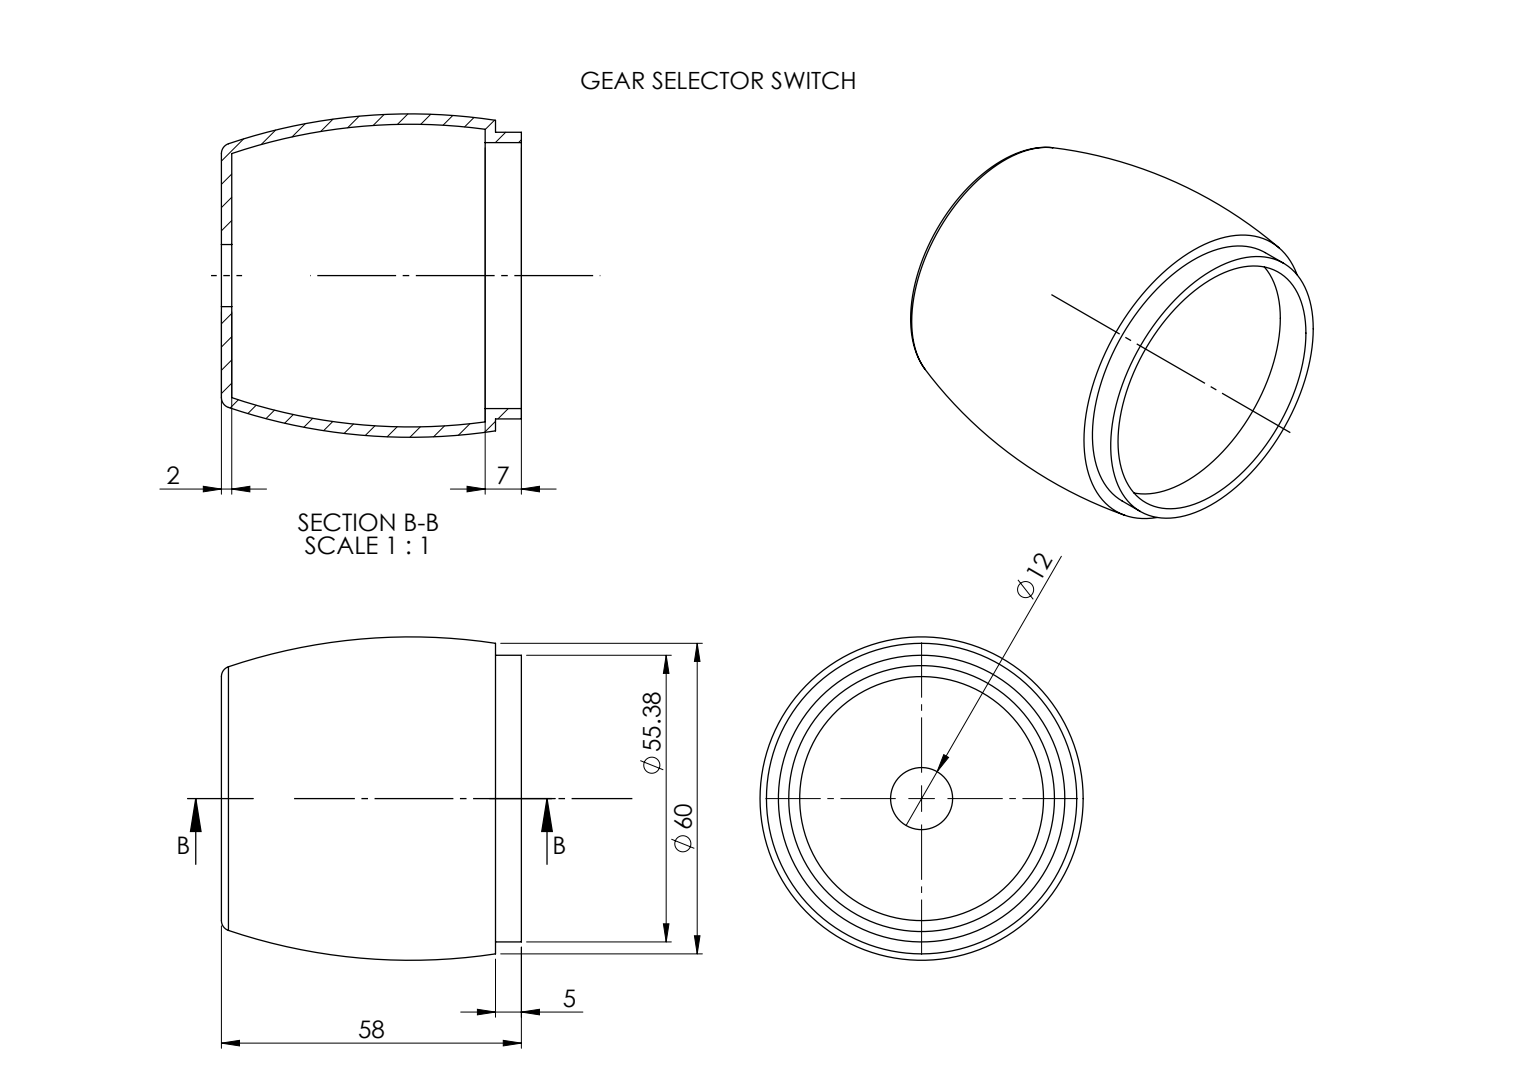
ISO-10303-21;
HEADER;
FILE_DESCRIPTION (('STEP AP214'),
    '1' );
FILE_NAME ('gear selector switch.step',
    '2026-10-05T20:22:16',
    ( '' ),
    ( '' ),
    'SwSTEP 2.0',
    'SolidWorks 2026',
    '' );
FILE_SCHEMA (( 'AUTOMOTIVE_DESIGN' ));
ENDSEC;

DATA;
#4=DIRECTION ( 'NONE',  ( 0.000000000000000000, 0.000000000000000000, -1.000000000000000000 ) ) ;
#45=ORIENTED_EDGE ( 'NONE', *, *, #7953, .F. ) ;
#49=PRODUCT_DEFINITION ( 'UNKNOWN', '', #15196, #232 ) ;
#123=PLANE ( 'NONE',  #15795 ) ;
#134=VERTEX_POINT ( 'NONE', #6129 ) ;
#138=ADVANCED_FACE ( 'NONE', ( #7376, #14017 ), #15677, .T. ) ;
#146=EDGE_CURVE ( 'NONE', #17383, #9593, #6108, .T. ) ;
#205=LINE ( 'NONE', #13586, #10347 ) ;
#217=SHAPE_DEFINITION_REPRESENTATION ( #9683, #10772 ) ;
#232=PRODUCT_DEFINITION_CONTEXT ( 'detailed design', #10711, 'design' ) ;
#249=FILL_AREA_STYLE_COLOUR ( '', #15123 ) ;
#272=CIRCLE ( 'NONE', #13562, 28.26633746182136164 ) ;
#285=DIRECTION ( 'NONE',  ( 0.000000000000000000, 0.000000000000000000, -1.000000000000000000 ) ) ;
#287=CIRCLE ( 'NONE', #5084, 23.57392898041429774 ) ;
#308=PLANE ( 'NONE',  #8782 ) ;
#348=CARTESIAN_POINT ( 'NONE',  ( -116.4755503550297107, 171.6227766016838245, 0.000000000000000000 ) ) ;
#409=AXIS2_PLACEMENT_3D ( 'NONE', #3562, #17022, #2059 ) ;
#411=ORIENTED_EDGE ( 'NONE', *, *, #16163, .T. ) ;
#425=ADVANCED_FACE ( 'NONE', ( #5501 ), #4977, .T. ) ;
#430=MECHANICAL_DESIGN_GEOMETRIC_PRESENTATION_REPRESENTATION('',(#7494),#12593);
#459=CARTESIAN_POINT ( 'NONE',  ( -95.00000000000000000, 171.6227766016838245, 0.000000000000000000 ) ) ;
#475=AXIS2_PLACEMENT_3D ( 'NONE', #11596, #1866, #6196 ) ;
#499=EDGE_CURVE ( 'NONE', #9593, #12318, #8101, .T. ) ;
#514=CYLINDRICAL_SURFACE ( 'NONE', #16412, 6.000000000000005329 ) ;
#554=VERTEX_POINT ( 'NONE', #15318 ) ;
#641=CARTESIAN_POINT ( 'NONE',  ( -153.0000000000000284, 171.6227766016838245, 0.000000000000000000 ) ) ;
#646=DIRECTION ( 'NONE',  ( 0.000000000000000000, 0.000000000000000000, 1.000000000000000000 ) ) ;
#675=SHAPE_REPRESENTATION_RELATIONSHIP ( 'NONE' , 'NONE' ,  #10772, #1721 ) ;
#691=CARTESIAN_POINT ( 'NONE',  ( -103.0000000000000142, 171.6227766016838245, 0.000000000000000000 ) ) ;
#724=CARTESIAN_POINT ( 'NONE',  ( -102.0000000000000142, 201.6227766016838245, 0.000000000000000000 ) ) ;
#743=AXIS2_PLACEMENT_3D ( 'NONE', #8605, #17020, #646 ) ;
#785=AXIS2_PLACEMENT_3D ( 'NONE', #9707, #16108, #10859 ) ;
#787=VECTOR ( 'NONE', #3451, 1000.000000000000000 ) ;
#893=ADVANCED_FACE ( 'NONE', ( #4594 ), #514, .F. ) ;
#959=ORIENTED_EDGE ( 'NONE', *, *, #13344, .T. ) ;
#972=DIRECTION ( 'NONE',  ( -0.000000000000000000, 0.000000000000000000, -1.000000000000000000 ) ) ;
#985=AXIS2_PLACEMENT_3D ( 'NONE', #17428, #10947, #13359 ) ;
#996=ORIENTED_EDGE ( 'NONE', *, *, #2991, .F. ) ;
#1026=TOROIDAL_SURFACE ( 'NONE', #8943, -78.75916623668499028, 108.0000000000000142 ) ;
#1028=CIRCLE ( 'NONE', #3301, 2.000000000000001776 ) ;
#1036=VERTEX_POINT ( 'NONE', #6706 ) ;
#1137=ORIENTED_EDGE ( 'NONE', *, *, #8044, .F. ) ;
#1138=CARTESIAN_POINT ( 'NONE',  ( -103.0000000000000142, 171.6227766016838245, 0.000000000000000000 ) ) ;
#1225=FACE_OUTER_BOUND ( 'NONE', #4522, .T. ) ;
#1270=AXIS2_PLACEMENT_3D ( 'NONE', #12415, #2602, #285 ) ;
#1280=PRODUCT_CONTEXT ( 'NONE', #3711, 'mechanical' ) ;
#1401=ADVANCED_FACE ( 'NONE', ( #15134 ), #11070, .F. ) ;
#1454=EDGE_CURVE ( 'NONE', #12318, #9593, #272, .T. ) ;
#1559=LINE ( 'NONE', #6964, #4454 ) ;
#1613=FACE_OUTER_BOUND ( 'NONE', #14014, .T. ) ;
#1631=VECTOR ( 'NONE', #13356, 1000.000000000000000 ) ;
#1699=DIRECTION ( 'NONE',  ( 0.000000000000000000, 0.000000000000000000, -1.000000000000000000 ) ) ;
#1707=PLANE ( 'NONE',  #14282 ) ;
#1714=CARTESIAN_POINT ( 'NONE',  ( -151.0000000000000284, 171.6227766016838245, 0.000000000000000000 ) ) ;
#1721=ADVANCED_BREP_SHAPE_REPRESENTATION ( '', ( #11363, #3583 ), #3025 ) ;
#1767=DIRECTION ( 'NONE',  ( 0.000000000000000000, 0.000000000000000000, -1.000000000000000000 ) ) ;
#1821=ORIENTED_EDGE ( 'NONE', *, *, #14197, .T. ) ;
#1836=PRESENTATION_STYLE_ASSIGNMENT (( #11217 ) ) ;
#1866=DIRECTION ( 'NONE',  ( 1.000000000000000000, -0.000000000000000000, -0.000000000000000000 ) ) ;
#1867=ADVANCED_FACE ( 'NONE', ( #5019, #10412 ), #123, .T. ) ;
#1901=CARTESIAN_POINT ( 'NONE',  ( -103.0000000000000142, 171.6227766016838245, 25.69059892324149175 ) ) ;
#1911=ORIENTED_EDGE ( 'NONE', *, *, #8044, .T. ) ;
#1914=FILL_AREA_STYLE_COLOUR ( '', #12928 ) ;
#1994=ORIENTED_EDGE ( 'NONE', *, *, #13315, .T. ) ;
#2031=CARTESIAN_POINT ( 'NONE',  ( -95.00000000000000000, 171.6227766016838245, 27.69059892324149530 ) ) ;
#2035=ORIENTED_EDGE ( 'NONE', *, *, #16198, .F. ) ;
#2059=DIRECTION ( 'NONE',  ( 0.000000000000000000, 0.000000000000000000, 1.000000000000000000 ) ) ;
#2068=DIRECTION ( 'NONE',  ( 0.000000000000000000, 0.000000000000000000, -1.000000000000000000 ) ) ;
#2111=CIRCLE ( 'NONE', #5222, 108.0000000000000142 ) ;
#2139=DIRECTION ( 'NONE',  ( -1.000000000000000000, 0.000000000000000000, 0.000000000000000000 ) ) ;
#2177=CARTESIAN_POINT ( 'NONE',  ( -95.00000000000000000, 171.6227766016838245, -25.69059892324149175 ) ) ;
#2190=CARTESIAN_POINT ( 'NONE',  ( -103.0000000000000142, 171.6227766016838245, -25.69059892324149175 ) ) ;
#2191=AXIS2_PLACEMENT_3D ( 'NONE', #4347, #13833, #1699 ) ;
#2195=VERTEX_POINT ( 'NONE', #9129 ) ;
#2227=DIRECTION ( 'NONE',  ( 0.000000000000000000, 0.000000000000000000, 1.000000000000000000 ) ) ;
#2275=EDGE_LOOP ( 'NONE', ( #10294, #17016, #12234, #9716 ) ) ;
#2291=VERTEX_POINT ( 'NONE', #16146 ) ;
#2361=ORIENTED_EDGE ( 'NONE', *, *, #7591, .T. ) ;
#2375=TOROIDAL_SURFACE ( 'NONE', #9156, -78.75916623668499028, 110.0000000000000142 ) ;
#2446=CIRCLE ( 'NONE', #14895, 27.69059892324149530 ) ;
#2461=STYLED_ITEM ( 'NONE', ( #16877 ), #1721 ) ;
#2472=AXIS2_PLACEMENT_3D ( 'NONE', #5028, #10419, #9274 ) ;
#2501=CIRCLE ( 'NONE', #10408, 6.000000000000005329 ) ;
#2600=ORIENTED_EDGE ( 'NONE', *, *, #3605, .T. ) ;
#2602=DIRECTION ( 'NONE',  ( 1.000000000000000000, -0.000000000000000000, -0.000000000000000000 ) ) ;
#2682=DIRECTION ( 'NONE',  ( 0.000000000000000000, 0.000000000000000000, -1.000000000000000000 ) ) ;
#2721=( NAMED_UNIT ( * ) SI_UNIT ( $, .STERADIAN. ) SOLID_ANGLE_UNIT ( ) );
#2726=EDGE_CURVE ( 'NONE', #5242, #10626, #4773, .T. ) ;
#2737=DIRECTION ( 'NONE',  ( 0.000000000000000000, 0.000000000000000000, -1.000000000000000000 ) ) ;
#2763=EDGE_LOOP ( 'NONE', ( #17460, #14468, #9016, #6481 ) ) ;
#2816=AXIS2_PLACEMENT_3D ( 'NONE', #9799, #14938, #5735 ) ;
#2846=ADVANCED_FACE ( 'NONE', ( #15997 ), #8199, .T. ) ;
#2855=CYLINDRICAL_SURFACE ( 'NONE', #1270, 6.000000000000005329 ) ;
#2928=ORIENTED_EDGE ( 'NONE', *, *, #2726, .T. ) ;
#2942=ORIENTED_EDGE ( 'NONE', *, *, #16368, .F. ) ;
#2991=EDGE_CURVE ( 'NONE', #15814, #10603, #9332, .T. ) ;
#3014=DIRECTION ( 'NONE',  ( 0.000000000000000000, 0.000000000000000000, -1.000000000000000000 ) ) ;
#3021=CARTESIAN_POINT ( 'NONE',  ( -100.0000000000000000, 171.6227766016838245, 0.000000000000000000 ) ) ;
#3025=( GEOMETRIC_REPRESENTATION_CONTEXT ( 3 ) GLOBAL_UNCERTAINTY_ASSIGNED_CONTEXT ( ( #7361 ) ) GLOBAL_UNIT_ASSIGNED_CONTEXT ( ( #7140, #5383, #2721 ) ) REPRESENTATION_CONTEXT ( 'NONE', 'WORKASPACE' ) );
#3197=PRODUCT ( 'gear selector switch', 'gear selector switch', '', ( #1280 ) ) ;
#3233=CIRCLE ( 'NONE', #409, 23.57392898041431195 ) ;
#3301=AXIS2_PLACEMENT_3D ( 'NONE', #3612, #10794, #2737 ) ;
#3322=EDGE_CURVE ( 'NONE', #8608, #3610, #10467, .T. ) ;
#3356=ORIENTED_EDGE ( 'NONE', *, *, #7036, .F. ) ;
#3357=DIRECTION ( 'NONE',  ( 1.000000000000000000, -0.000000000000000000, -0.000000000000000000 ) ) ;
#3408=DIRECTION ( 'NONE',  ( 1.000000000000000000, -0.000000000000000000, -0.000000000000000000 ) ) ;
#3414=DIRECTION ( 'NONE',  ( -1.000000000000000000, 0.000000000000000000, 0.000000000000000000 ) ) ;
#3423=ADVANCED_FACE ( 'NONE', ( #5710, #10918 ), #308, .F. ) ;
#3451=DIRECTION ( 'NONE',  ( 1.000000000000000000, -0.000000000000000000, -0.000000000000000000 ) ) ;
#3522=AXIS2_PLACEMENT_3D ( 'NONE', #9734, #5760, #3014 ) ;
#3562=CARTESIAN_POINT ( 'NONE',  ( -153.0000000000000284, 171.6227766016838245, 0.000000000000000000 ) ) ;
#3583=AXIS2_PLACEMENT_3D ( 'NONE', #5482, #6893, #8222 ) ;
#3605=EDGE_CURVE ( 'NONE', #1036, #16730, #8421, .T. ) ;
#3610=VERTEX_POINT ( 'NONE', #7874 ) ;
#3612=CARTESIAN_POINT ( 'NONE',  ( -151.0000000000000284, 171.6227766016838245, 23.57392898041431195 ) ) ;
#3641=CARTESIAN_POINT ( 'NONE',  ( -100.0000000000000000, 171.6227766016838245, 30.00000000000000711 ) ) ;
#3711=APPLICATION_CONTEXT ( 'automotive_design' ) ;
#3712=DIRECTION ( 'NONE',  ( 1.000000000000000000, -0.000000000000000000, -0.000000000000000000 ) ) ;
#3756=EDGE_LOOP ( 'NONE', ( #14052, #411 ) ) ;
#3813=CARTESIAN_POINT ( 'NONE',  ( -103.0000000000000142, 171.6227766016838245, 0.000000000000000000 ) ) ;
#3889=DIRECTION ( 'NONE',  ( 1.000000000000000000, -0.000000000000000000, -0.000000000000000000 ) ) ;
#3895=AXIS2_PLACEMENT_3D ( 'NONE', #1138, #3889, #14500 ) ;
#4041=CARTESIAN_POINT ( 'NONE',  ( -116.4755503550297107, 171.6227766016838245, 78.75916623668499028 ) ) ;
#4069=ORIENTED_EDGE ( 'NONE', *, *, #5991, .T. ) ;
#4091=DIRECTION ( 'NONE',  ( 0.000000000000000000, 0.000000000000000000, -1.000000000000000000 ) ) ;
#4106=ORIENTED_EDGE ( 'NONE', *, *, #16368, .T. ) ;
#4108=DIRECTION ( 'NONE',  ( 1.000000000000000000, -0.000000000000000000, -0.000000000000000000 ) ) ;
#4111=ORIENTED_EDGE ( 'NONE', *, *, #13315, .F. ) ;
#4129=EDGE_LOOP ( 'NONE', ( #4653, #5827 ) ) ;
#4176=DIRECTION ( 'NONE',  ( 1.000000000000000000, -0.000000000000000000, -0.000000000000000000 ) ) ;
#4209=DIRECTION ( 'NONE',  ( 0.000000000000000000, 0.000000000000000000, 1.000000000000000000 ) ) ;
#4267=DIRECTION ( 'NONE',  ( 0.000000000000000000, 0.000000000000000000, -1.000000000000000000 ) ) ;
#4268=EDGE_LOOP ( 'NONE', ( #12681, #16145 ) ) ;
#4347=CARTESIAN_POINT ( 'NONE',  ( -103.0000000000000142, 171.6227766016838245, 0.000000000000000000 ) ) ;
#4354=AXIS2_PLACEMENT_3D ( 'NONE', #4478, #3408, #2068 ) ;
#4361=DIRECTION ( 'NONE',  ( 0.000000000000000000, 0.000000000000000000, -1.000000000000000000 ) ) ;
#4363=ORIENTED_EDGE ( 'NONE', *, *, #146, .F. ) ;
#4454=VECTOR ( 'NONE', #12364, 1000.000000000000000 ) ;
#4478=CARTESIAN_POINT ( 'NONE',  ( -95.00000000000000000, 171.6227766016838245, 0.000000000000000000 ) ) ;
#4522=EDGE_LOOP ( 'NONE', ( #13245, #15418, #16764, #6931 ) ) ;
#4540=DIRECTION ( 'NONE',  ( 1.000000000000000000, -0.000000000000000000, -0.000000000000000000 ) ) ;
#4541=CIRCLE ( 'NONE', #5390, 110.0000000000000142 ) ;
#4594=FACE_OUTER_BOUND ( 'NONE', #16314, .T. ) ;
#4615=DIRECTION ( 'NONE',  ( 1.000000000000000000, -0.000000000000000000, -0.000000000000000000 ) ) ;
#4653=ORIENTED_EDGE ( 'NONE', *, *, #10399, .T. ) ;
#4702=AXIS2_PLACEMENT_3D ( 'NONE', #10035, #3414, #16785 ) ;
#4739=FACE_BOUND ( 'NONE', #6262, .T. ) ;
#4768=ORIENTED_EDGE ( 'NONE', *, *, #15114, .T. ) ;
#4769=DIRECTION ( 'NONE',  ( 1.000000000000000000, -0.000000000000000000, -0.000000000000000000 ) ) ;
#4773=LINE ( 'NONE', #2190, #16125 ) ;
#4778=CIRCLE ( 'NONE', #5347, 30.00000000000000000 ) ;
#4834=ORIENTED_EDGE ( 'NONE', *, *, #10792, .F. ) ;
#4845=ADVANCED_FACE ( 'NONE', ( #5510 ), #2855, .F. ) ;
#4848=CARTESIAN_POINT ( 'NONE',  ( -116.4755503550297107, 171.6227766016838245, -78.75916623668499028 ) ) ;
#4854=DIRECTION ( 'NONE',  ( 0.000000000000000000, 0.000000000000000000, -1.000000000000000000 ) ) ;
#4914=CARTESIAN_POINT ( 'NONE',  ( -153.0000000000000284, 171.6227766016838245, 6.000000000000005329 ) ) ;
#4925=EDGE_CURVE ( 'NONE', #2195, #554, #10302, .T. ) ;
#4977=TOROIDAL_SURFACE ( 'NONE', #9498, -78.75916623668499028, 110.0000000000000142 ) ;
#4996=ADVANCED_FACE ( 'NONE', ( #11347, #7365 ), #1707, .F. ) ;
#5019=FACE_OUTER_BOUND ( 'NONE', #8020, .T. ) ;
#5028=CARTESIAN_POINT ( 'NONE',  ( -102.0000000000000142, 171.6227766016838245, 0.000000000000000000 ) ) ;
#5084=AXIS2_PLACEMENT_3D ( 'NONE', #16995, #3712, #9096 ) ;
#5121=VERTEX_POINT ( 'NONE', #3641 ) ;
#5127=DIRECTION ( 'NONE',  ( 0.000000000000000000, 0.000000000000000000, -1.000000000000000000 ) ) ;
#5146=DIRECTION ( 'NONE',  ( 1.000000000000000000, -0.000000000000000000, -0.000000000000000000 ) ) ;
#5171=EDGE_LOOP ( 'NONE', ( #6592, #2361, #16013, #15183 ) ) ;
#5222=AXIS2_PLACEMENT_3D ( 'NONE', #12160, #8164, #12417 ) ;
#5242=VERTEX_POINT ( 'NONE', #12013 ) ;
#5246=VERTEX_POINT ( 'NONE', #17147 ) ;
#5302=DIRECTION ( 'NONE',  ( 1.000000000000000000, -0.000000000000000000, -0.000000000000000000 ) ) ;
#5347=AXIS2_PLACEMENT_3D ( 'NONE', #12562, #16738, #9906 ) ;
#5383=( NAMED_UNIT ( * ) PLANE_ANGLE_UNIT ( ) SI_UNIT ( $, .RADIAN. ) );
#5390=AXIS2_PLACEMENT_3D ( 'NONE', #4848, #14229, #7578 ) ;
#5482=CARTESIAN_POINT ( 'NONE',  ( 0.000000000000000000, 0.000000000000000000, 0.000000000000000000 ) ) ;
#5501=FACE_OUTER_BOUND ( 'NONE', #5171, .T. ) ;
#5510=FACE_OUTER_BOUND ( 'NONE', #9230, .T. ) ;
#5520=DIRECTION ( 'NONE',  ( 0.000000000000000000, 0.000000000000000000, -1.000000000000000000 ) ) ;
#5560=CARTESIAN_POINT ( 'NONE',  ( -95.00000000000000000, 171.6227766016838245, 25.69059892324149175 ) ) ;
#5563=FILL_AREA_STYLE ('',( #249 ) ) ;
#5644=DIRECTION ( 'NONE',  ( 1.000000000000000000, -0.000000000000000000, -0.000000000000000000 ) ) ;
#5710=FACE_BOUND ( 'NONE', #4268, .T. ) ;
#5735=DIRECTION ( 'NONE',  ( 0.000000000000000000, 0.000000000000000000, -1.000000000000000000 ) ) ;
#5760=DIRECTION ( 'NONE',  ( 1.000000000000000000, -0.000000000000000000, -0.000000000000000000 ) ) ;
#5827=ORIENTED_EDGE ( 'NONE', *, *, #2991, .T. ) ;
#5897=ORIENTED_EDGE ( 'NONE', *, *, #14197, .F. ) ;
#5912=CARTESIAN_POINT ( 'NONE',  ( -153.0000000000000284, 171.6227766016838245, -6.000000000000005329 ) ) ;
#5968=CARTESIAN_POINT ( 'NONE',  ( -151.0000000000000284, 171.6227766016838245, -23.57392898041431195 ) ) ;
#5985=FACE_OUTER_BOUND ( 'NONE', #10484, .T. ) ;
#5991=EDGE_CURVE ( 'NONE', #17383, #134, #15147, .T. ) ;
#5994=ORIENTED_EDGE ( 'NONE', *, *, #7134, .T. ) ;
#6034=ADVANCED_FACE ( 'NONE', ( #1613 ), #1026, .F. ) ;
#6085=DIRECTION ( 'NONE',  ( 0.000000000000000000, 0.000000000000000000, -1.000000000000000000 ) ) ;
#6108=CIRCLE ( 'NONE', #743, 108.0000000000000142 ) ;
#6117=DIRECTION ( 'NONE',  ( 1.000000000000000000, 0.000000000000000000, -0.000000000000000000 ) ) ;
#6129=CARTESIAN_POINT ( 'NONE',  ( -151.0000000000000284, 171.6227766016838245, -23.57392898041429774 ) ) ;
#6153=CIRCLE ( 'NONE', #2472, 25.69059892324149175 ) ;
#6177=CARTESIAN_POINT ( 'NONE',  ( -95.00000000000000000, 171.6227766016838245, 0.000000000000000000 ) ) ;
#6196=DIRECTION ( 'NONE',  ( 0.000000000000000000, 0.000000000000000000, -1.000000000000000000 ) ) ;
#6214=ADVANCED_FACE ( 'NONE', ( #15328 ), #16019, .F. ) ;
#6262=EDGE_LOOP ( 'NONE', ( #16312, #5897 ) ) ;
#6314=ORIENTED_EDGE ( 'NONE', *, *, #16708, .T. ) ;
#6337=DIRECTION ( 'NONE',  ( -0.000000000000000000, 0.000000000000000000, -1.000000000000000000 ) ) ;
#6342=CARTESIAN_POINT ( 'NONE',  ( -151.0000000000000284, 171.6227766016838245, 0.000000000000000000 ) ) ;
#6355=AXIS2_PLACEMENT_3D ( 'NONE', #16114, #5302, #5127 ) ;
#6411=CIRCLE ( 'NONE', #475, 30.00000000000000000 ) ;
#6481=ORIENTED_EDGE ( 'NONE', *, *, #17060, .F. ) ;
#6505=UNCERTAINTY_MEASURE_WITH_UNIT (LENGTH_MEASURE( 1.000000000000000082E-05 ), #6976, 'distance_accuracy_value', 'NONE');
#6563=CARTESIAN_POINT ( 'NONE',  ( -151.6393416600920716, 171.6227766016838245, 0.000000000000000000 ) ) ;
#6574=ORIENTED_EDGE ( 'NONE', *, *, #7591, .F. ) ;
#6592=ORIENTED_EDGE ( 'NONE', *, *, #8483, .F. ) ;
#6634=AXIS2_PLACEMENT_3D ( 'NONE', #5968, #15679, #12857 ) ;
#6706=CARTESIAN_POINT ( 'NONE',  ( -151.0000000000000284, 171.6227766016838245, -6.000000000000005329 ) ) ;
#6764=ADVANCED_FACE ( 'NONE', ( #8494 ), #2375, .T. ) ;
#6881=VERTEX_POINT ( 'NONE', #14240 ) ;
#6885=SURFACE_STYLE_FILL_AREA ( #5563 ) ;
#6893=DIRECTION ( 'NONE',  ( 0.000000000000000000, 0.000000000000000000, 1.000000000000000000 ) ) ;
#6930=TOROIDAL_SURFACE ( 'NONE', #985, 23.57392898041431195, 2.000000000000000000 ) ;
#6931=ORIENTED_EDGE ( 'NONE', *, *, #16757, .F. ) ;
#6939=DIRECTION ( 'NONE',  ( 0.000000000000000000, 0.000000000000000000, -1.000000000000000000 ) ) ;
#6964=CARTESIAN_POINT ( 'NONE',  ( -103.0000000000000142, 171.6227766016838245, -27.69059892324149530 ) ) ;
#6967=CARTESIAN_POINT ( 'NONE',  ( -153.0000000000000284, 171.6227766016838245, 0.000000000000000000 ) ) ;
#6969=AXIS2_PLACEMENT_3D ( 'NONE', #13565, #13646, #4267 ) ;
#6976=( LENGTH_UNIT ( ) NAMED_UNIT ( * ) SI_UNIT ( .MILLI., .METRE. ) );
#7036=EDGE_CURVE ( 'NONE', #16418, #10459, #12868, .T. ) ;
#7093=DIRECTION ( 'NONE',  ( 1.000000000000000000, -0.000000000000000000, -0.000000000000000000 ) ) ;
#7104=DIRECTION ( 'NONE',  ( 0.000000000000000000, 0.000000000000000000, 1.000000000000000000 ) ) ;
#7134=EDGE_CURVE ( 'NONE', #10459, #10626, #11983, .T. ) ;
#7140=( LENGTH_UNIT ( ) NAMED_UNIT ( * ) SI_UNIT ( .MILLI., .METRE. ) );
#7208=EDGE_CURVE ( 'NONE', #134, #12318, #2111, .T. ) ;
#7244=ORIENTED_EDGE ( 'NONE', *, *, #3322, .F. ) ;
#7313=SURFACE_SIDE_STYLE ('',( #10139 ) ) ;
#7361=UNCERTAINTY_MEASURE_WITH_UNIT (LENGTH_MEASURE( 1.000000000000000082E-05 ), #7140, 'distance_accuracy_value', 'NONE');
#7365=FACE_BOUND ( 'NONE', #15473, .T. ) ;
#7375=DIRECTION ( 'NONE',  ( 1.000000000000000000, -0.000000000000000000, -0.000000000000000000 ) ) ;
#7376=FACE_OUTER_BOUND ( 'NONE', #3756, .T. ) ;
#7469=EDGE_LOOP ( 'NONE', ( #4768, #13782 ) ) ;
#7477=SURFACE_STYLE_USAGE ( .BOTH. , #7313 ) ;
#7494=STYLED_ITEM ( 'NONE', ( #1836 ), #11363 ) ;
#7552=DIRECTION ( 'NONE',  ( 1.000000000000000000, -0.000000000000000000, -0.000000000000000000 ) ) ;
#7578=DIRECTION ( 'NONE',  ( 0.000000000000000000, 0.000000000000000000, 1.000000000000000000 ) ) ;
#7591=EDGE_CURVE ( 'NONE', #10629, #8608, #13415, .T. ) ;
#7644=ADVANCED_FACE ( 'NONE', ( #11769 ), #17180, .T. ) ;
#7673=ORIENTED_EDGE ( 'NONE', *, *, #9928, .T. ) ;
#7739=ORIENTED_EDGE ( 'NONE', *, *, #16359, .T. ) ;
#7874=CARTESIAN_POINT ( 'NONE',  ( -100.0000000000000000, 171.6227766016838245, -30.00000000000000711 ) ) ;
#7951=CARTESIAN_POINT ( 'NONE',  ( -103.0000000000000142, 171.6227766016838245, 6.000000000000005329 ) ) ;
#7953=EDGE_CURVE ( 'NONE', #10603, #1036, #9011, .T. ) ;
#7955=FACE_OUTER_BOUND ( 'NONE', #8436, .T. ) ;
#8020=EDGE_LOOP ( 'NONE', ( #8586, #7673 ) ) ;
#8044=EDGE_CURVE ( 'NONE', #134, #17383, #287, .T. ) ;
#8070=DIRECTION ( 'NONE',  ( 1.000000000000000000, -0.000000000000000000, -0.000000000000000000 ) ) ;
#8101=CIRCLE ( 'NONE', #6969, 28.26633746182136164 ) ;
#8164=DIRECTION ( 'NONE',  ( -0.000000000000000000, -1.000000000000000000, -0.000000000000000000 ) ) ;
#8199=TOROIDAL_SURFACE ( 'NONE', #16690, 23.57392898041431195, 2.000000000000000000 ) ;
#8222=DIRECTION ( 'NONE',  ( 1.000000000000000000, 0.000000000000000000, 0.000000000000000000 ) ) ;
#8331=DIRECTION ( 'NONE',  ( -1.000000000000000000, 0.000000000000000000, 0.000000000000000000 ) ) ;
#8414=CARTESIAN_POINT ( 'NONE',  ( -151.6393416600920716, 171.6227766016838245, 0.000000000000000000 ) ) ;
#8421=CIRCLE ( 'NONE', #12955, 6.000000000000005329 ) ;
#8436=EDGE_LOOP ( 'NONE', ( #2035, #6574, #6314, #11975 ) ) ;
#8483=EDGE_CURVE ( 'NONE', #10629, #5121, #4541, .T. ) ;
#8494=FACE_OUTER_BOUND ( 'NONE', #10932, .T. ) ;
#8553=( NAMED_UNIT ( * ) PLANE_ANGLE_UNIT ( ) SI_UNIT ( $, .RADIAN. ) );
#8586=ORIENTED_EDGE ( 'NONE', *, *, #16428, .T. ) ;
#8588=CARTESIAN_POINT ( 'NONE',  ( -102.0000000000000142, 171.6227766016838245, 0.000000000000000000 ) ) ;
#8605=CARTESIAN_POINT ( 'NONE',  ( -116.4755503550297107, 171.6227766016838245, -78.75916623668499028 ) ) ;
#8608=VERTEX_POINT ( 'NONE', #12263 ) ;
#8628=PLANE ( 'NONE',  #4702 ) ;
#8640=FILL_AREA_STYLE ('',( #1914 ) ) ;
#8668=DIRECTION ( 'NONE',  ( 1.000000000000000000, -0.000000000000000000, -0.000000000000000000 ) ) ;
#8676=ORIENTED_EDGE ( 'NONE', *, *, #1454, .T. ) ;
#8782=AXIS2_PLACEMENT_3D ( 'NONE', #11095, #16341, #4209 ) ;
#8943=AXIS2_PLACEMENT_3D ( 'NONE', #10819, #8070, #2682 ) ;
#9011=LINE ( 'NONE', #11747, #787 ) ;
#9016=ORIENTED_EDGE ( 'NONE', *, *, #15114, .F. ) ;
#9089=DIRECTION ( 'NONE',  ( 0.000000000000000000, 0.000000000000000000, 1.000000000000000000 ) ) ;
#9096=DIRECTION ( 'NONE',  ( 0.000000000000000000, 0.000000000000000000, -1.000000000000000000 ) ) ;
#9129=CARTESIAN_POINT ( 'NONE',  ( -100.0000000000000000, 171.6227766016838245, 27.69059892324149530 ) ) ;
#9156=AXIS2_PLACEMENT_3D ( 'NONE', #348, #8668, #1767 ) ;
#9173=AXIS2_PLACEMENT_3D ( 'NONE', #3813, #11679, #10353 ) ;
#9200=CARTESIAN_POINT ( 'NONE',  ( -102.0000000000000142, 171.6227766016838245, -28.26633746182137585 ) ) ;
#9230=EDGE_LOOP ( 'NONE', ( #10524, #15538, #11141, #2600 ) ) ;
#9274=DIRECTION ( 'NONE',  ( 0.000000000000000000, 0.000000000000000000, -1.000000000000000000 ) ) ;
#9332=CIRCLE ( 'NONE', #14165, 6.000000000000005329 ) ;
#9469=CARTESIAN_POINT ( 'NONE',  ( -116.4755503550297107, 171.6227766016838245, 0.000000000000000000 ) ) ;
#9498=AXIS2_PLACEMENT_3D ( 'NONE', #9469, #4176, #4091 ) ;
#9593=VERTEX_POINT ( 'NONE', #16321 ) ;
#9683=PRODUCT_DEFINITION_SHAPE ( 'NONE', 'NONE',  #49 ) ;
#9707=CARTESIAN_POINT ( 'NONE',  ( -100.0000000000000000, 171.6227766016838245, 0.000000000000000000 ) ) ;
#9716=ORIENTED_EDGE ( 'NONE', *, *, #7208, .F. ) ;
#9734=CARTESIAN_POINT ( 'NONE',  ( -102.0000000000000142, 171.6227766016838245, 0.000000000000000000 ) ) ;
#9755=CARTESIAN_POINT ( 'NONE',  ( -95.00000000000000000, 171.6227766016838245, 0.000000000000000000 ) ) ;
#9799=CARTESIAN_POINT ( 'NONE',  ( -153.0000000000000284, 171.6227766016838245, 0.000000000000000000 ) ) ;
#9855=ORIENTED_EDGE ( 'NONE', *, *, #4925, .F. ) ;
#9876=AXIS2_PLACEMENT_3D ( 'NONE', #459, #7375, #13851 ) ;
#9906=DIRECTION ( 'NONE',  ( 0.000000000000000000, 0.000000000000000000, -1.000000000000000000 ) ) ;
#9924=DIRECTION ( 'NONE',  ( 1.000000000000000000, -0.000000000000000000, -0.000000000000000000 ) ) ;
#9928=EDGE_CURVE ( 'NONE', #5121, #3610, #4778, .T. ) ;
#9974=DIRECTION ( 'NONE',  ( 1.000000000000000000, -0.000000000000000000, -0.000000000000000000 ) ) ;
#9993=DIRECTION ( 'NONE',  ( 0.000000000000000000, 0.000000000000000000, -1.000000000000000000 ) ) ;
#10035=CARTESIAN_POINT ( 'NONE',  ( -151.0000000000000284, 196.6227766016838245, 0.000000000000000000 ) ) ;
#10139=SURFACE_STYLE_FILL_AREA ( #8640 ) ;
#10260=CARTESIAN_POINT ( 'NONE',  ( -102.0000000000000142, 171.6227766016838245, 25.69059892324149175 ) ) ;
#10294=ORIENTED_EDGE ( 'NONE', *, *, #5991, .F. ) ;
#10302=CIRCLE ( 'NONE', #17101, 27.69059892324149530 ) ;
#10326=CLOSED_SHELL ( 'NONE', ( #2846, #6764, #7644, #1401, #6214, #893, #138, #4845, #11969, #6034, #4996, #13273, #3423, #11273, #1867, #425, #11243 ) ) ;
#10347=VECTOR ( 'NONE', #4108, 1000.000000000000000 ) ;
#10353=DIRECTION ( 'NONE',  ( 0.000000000000000000, 0.000000000000000000, -1.000000000000000000 ) ) ;
#10399=EDGE_CURVE ( 'NONE', #10603, #15814, #12146, .T. ) ;
#10408=AXIS2_PLACEMENT_3D ( 'NONE', #1714, #16676, #4361 ) ;
#10412=FACE_BOUND ( 'NONE', #14490, .T. ) ;
#10419=DIRECTION ( 'NONE',  ( 1.000000000000000000, -0.000000000000000000, -0.000000000000000000 ) ) ;
#10459=VERTEX_POINT ( 'NONE', #5560 ) ;
#10467=CIRCLE ( 'NONE', #11322, 110.0000000000000142 ) ;
#10484=EDGE_LOOP ( 'NONE', ( #1911, #4069 ) ) ;
#10521=ORIENTED_EDGE ( 'NONE', *, *, #16198, .T. ) ;
#10524=ORIENTED_EDGE ( 'NONE', *, *, #13344, .F. ) ;
#10535=ORIENTED_EDGE ( 'NONE', *, *, #16428, .F. ) ;
#10586=AXIS2_PLACEMENT_3D ( 'NONE', #6563, #5146, #11606 ) ;
#10595=FACE_OUTER_BOUND ( 'NONE', #13149, .T. ) ;
#10603=VERTEX_POINT ( 'NONE', #5912 ) ;
#10626=VERTEX_POINT ( 'NONE', #2177 ) ;
#10629=VERTEX_POINT ( 'NONE', #15632 ) ;
#10711=APPLICATION_CONTEXT ( 'automotive_design' ) ;
#10772=SHAPE_REPRESENTATION ( 'gear selector switch', ( #3583 ), #3025 ) ;
#10792=EDGE_CURVE ( 'NONE', #6881, #5246, #15968, .T. ) ;
#10794=DIRECTION ( 'NONE',  ( 0.000000000000000000, -1.000000000000000000, 0.000000000000000000 ) ) ;
#10819=CARTESIAN_POINT ( 'NONE',  ( -116.4755503550297107, 171.6227766016838245, 0.000000000000000000 ) ) ;
#10858=ORIENTED_EDGE ( 'NONE', *, *, #7036, .T. ) ;
#10859=DIRECTION ( 'NONE',  ( 0.000000000000000000, 0.000000000000000000, -1.000000000000000000 ) ) ;
#10918=FACE_OUTER_BOUND ( 'NONE', #7469, .T. ) ;
#10932=EDGE_LOOP ( 'NONE', ( #4106, #12016, #10535, #7244 ) ) ;
#10934=( GEOMETRIC_REPRESENTATION_CONTEXT ( 3 ) GLOBAL_UNCERTAINTY_ASSIGNED_CONTEXT ( ( #16919 ) ) GLOBAL_UNIT_ASSIGNED_CONTEXT ( ( #12805, #8553, #15286 ) ) REPRESENTATION_CONTEXT ( 'NONE', 'WORKASPACE' ) );
#10947=DIRECTION ( 'NONE',  ( -1.000000000000000000, 0.000000000000000000, 0.000000000000000000 ) ) ;
#11044=( NAMED_UNIT ( * ) SI_UNIT ( $, .STERADIAN. ) SOLID_ANGLE_UNIT ( ) );
#11070=CYLINDRICAL_SURFACE ( 'NONE', #2191, 25.69059892324149175 ) ;
#11095=CARTESIAN_POINT ( 'NONE',  ( -95.00000000000000000, 199.3133755249253056, 0.000000000000000000 ) ) ;
#11141=ORIENTED_EDGE ( 'NONE', *, *, #7953, .T. ) ;
#11142=CIRCLE ( 'NONE', #3522, 25.69059892324149175 ) ;
#11209=AXIS2_PLACEMENT_3D ( 'NONE', #14099, #9924, #16575 ) ;
#11217=SURFACE_STYLE_USAGE ( .BOTH. , #11311 ) ;
#11243=ADVANCED_FACE ( 'NONE', ( #7955 ), #6930, .T. ) ;
#11273=ADVANCED_FACE ( 'NONE', ( #1225 ), #11844, .T. ) ;
#11311=SURFACE_SIDE_STYLE ('',( #6885 ) ) ;
#11322=AXIS2_PLACEMENT_3D ( 'NONE', #4041, #16248, #6939 ) ;
#11347=FACE_OUTER_BOUND ( 'NONE', #12600, .T. ) ;
#11363=MANIFOLD_SOLID_BREP ( 'Fillet1', #10326 ) ;
#11515=CIRCLE ( 'NONE', #785, 27.69059892324149530 ) ;
#11596=CARTESIAN_POINT ( 'NONE',  ( -100.0000000000000000, 171.6227766016838245, 0.000000000000000000 ) ) ;
#11606=DIRECTION ( 'NONE',  ( 0.000000000000000000, 0.000000000000000000, -1.000000000000000000 ) ) ;
#11614=CARTESIAN_POINT ( 'NONE',  ( -153.0000000000000284, 196.6227766016838245, 0.000000000000000000 ) ) ;
#11679=DIRECTION ( 'NONE',  ( 1.000000000000000000, -0.000000000000000000, -0.000000000000000000 ) ) ;
#11686=ORIENTED_EDGE ( 'NONE', *, *, #16708, .F. ) ;
#11744=CYLINDRICAL_SURFACE ( 'NONE', #3895, 25.69059892324149175 ) ;
#11747=CARTESIAN_POINT ( 'NONE',  ( -103.0000000000000142, 171.6227766016838245, -6.000000000000005329 ) ) ;
#11769=FACE_OUTER_BOUND ( 'NONE', #2763, .T. ) ;
#11844=CYLINDRICAL_SURFACE ( 'NONE', #6355, 27.69059892324149530 ) ;
#11853=CARTESIAN_POINT ( 'NONE',  ( -151.0000000000000284, 171.6227766016838245, 23.57392898041429774 ) ) ;
#11969=ADVANCED_FACE ( 'NONE', ( #4739, #5985 ), #8628, .F. ) ;
#11975=ORIENTED_EDGE ( 'NONE', *, *, #16163, .F. ) ;
#11983=CIRCLE ( 'NONE', #4354, 25.69059892324149175 ) ;
#11998=CIRCLE ( 'NONE', #6634, 2.000000000000001776 ) ;
#12013=CARTESIAN_POINT ( 'NONE',  ( -102.0000000000000142, 171.6227766016838245, -25.69059892324149175 ) ) ;
#12016=ORIENTED_EDGE ( 'NONE', *, *, #8483, .T. ) ;
#12146=CIRCLE ( 'NONE', #2816, 6.000000000000005329 ) ;
#12160=CARTESIAN_POINT ( 'NONE',  ( -116.4755503550297107, 171.6227766016838245, 78.75916623668499028 ) ) ;
#12199=EDGE_CURVE ( 'NONE', #10626, #10459, #16007, .T. ) ;
#12234=ORIENTED_EDGE ( 'NONE', *, *, #499, .T. ) ;
#12250=EDGE_CURVE ( 'NONE', #2195, #13060, #205, .T. ) ;
#12263=CARTESIAN_POINT ( 'NONE',  ( -151.6393416600920716, 171.6227766016838245, -25.46898629924947244 ) ) ;
#12318=VERTEX_POINT ( 'NONE', #9200 ) ;
#12325=AXIS2_PLACEMENT_3D ( 'NONE', #11614, #2139, #2227 ) ;
#12364=DIRECTION ( 'NONE',  ( 1.000000000000000000, -0.000000000000000000, -0.000000000000000000 ) ) ;
#12415=CARTESIAN_POINT ( 'NONE',  ( -103.0000000000000142, 171.6227766016838245, 0.000000000000000000 ) ) ;
#12417=DIRECTION ( 'NONE',  ( 0.000000000000000000, 0.000000000000000000, -1.000000000000000000 ) ) ;
#12494=DIRECTION ( 'NONE',  ( 0.000000000000000000, 0.000000000000000000, -1.000000000000000000 ) ) ;
#12562=CARTESIAN_POINT ( 'NONE',  ( -100.0000000000000000, 171.6227766016838245, 0.000000000000000000 ) ) ;
#12593=( GEOMETRIC_REPRESENTATION_CONTEXT ( 3 ) GLOBAL_UNCERTAINTY_ASSIGNED_CONTEXT ( ( #6505 ) ) GLOBAL_UNIT_ASSIGNED_CONTEXT ( ( #6976, #16725, #11044 ) ) REPRESENTATION_CONTEXT ( 'NONE', 'WORKASPACE' ) );
#12600=EDGE_LOOP ( 'NONE', ( #13117, #13200 ) ) ;
#12681=ORIENTED_EDGE ( 'NONE', *, *, #12199, .F. ) ;
#12712=ORIENTED_EDGE ( 'NONE', *, *, #2726, .F. ) ;
#12805=( LENGTH_UNIT ( ) NAMED_UNIT ( * ) SI_UNIT ( .MILLI., .METRE. ) );
#12857=DIRECTION ( 'NONE',  ( 0.000000000000000000, 0.000000000000000000, 1.000000000000000000 ) ) ;
#12868=LINE ( 'NONE', #1901, #17369 ) ;
#12928=COLOUR_RGB ( '', 0.66274510, 0.83137255, 0.94901961) ;
#12955=AXIS2_PLACEMENT_3D ( 'NONE', #14701, #13455, #4 ) ;
#13007=LINE ( 'NONE', #7951, #1631 ) ;
#13036=ORIENTED_EDGE ( 'NONE', *, *, #12199, .T. ) ;
#13060=VERTEX_POINT ( 'NONE', #2031 ) ;
#13117=ORIENTED_EDGE ( 'NONE', *, *, #1454, .F. ) ;
#13149=EDGE_LOOP ( 'NONE', ( #3356, #4111, #2928, #13036 ) ) ;
#13200=ORIENTED_EDGE ( 'NONE', *, *, #499, .F. ) ;
#13245=ORIENTED_EDGE ( 'NONE', *, *, #12250, .F. ) ;
#13273=ADVANCED_FACE ( 'NONE', ( #10595 ), #11744, .F. ) ;
#13315=EDGE_CURVE ( 'NONE', #5242, #16418, #6153, .T. ) ;
#13344=EDGE_CURVE ( 'NONE', #15814, #16730, #13007, .T. ) ;
#13349=CARTESIAN_POINT ( 'NONE',  ( -100.0000000000000000, 201.6227766016838245, 0.000000000000000000 ) ) ;
#13356=DIRECTION ( 'NONE',  ( 1.000000000000000000, -0.000000000000000000, -0.000000000000000000 ) ) ;
#13359=DIRECTION ( 'NONE',  ( 0.000000000000000000, 0.000000000000000000, 1.000000000000000000 ) ) ;
#13365=ORIENTED_EDGE ( 'NONE', *, *, #7208, .T. ) ;
#13382=EDGE_LOOP ( 'NONE', ( #17121, #10858, #5994, #12712 ) ) ;
#13390=EDGE_CURVE ( 'NONE', #554, #2195, #11515, .T. ) ;
#13415=CIRCLE ( 'NONE', #10586, 25.46898629924947244 ) ;
#13419=AXIS2_PLACEMENT_3D ( 'NONE', #8414, #7093, #12494 ) ;
#13455=DIRECTION ( 'NONE',  ( 1.000000000000000000, -0.000000000000000000, -0.000000000000000000 ) ) ;
#13562=AXIS2_PLACEMENT_3D ( 'NONE', #8588, #4615, #9993 ) ;
#13565=CARTESIAN_POINT ( 'NONE',  ( -102.0000000000000142, 171.6227766016838245, 0.000000000000000000 ) ) ;
#13586=CARTESIAN_POINT ( 'NONE',  ( -103.0000000000000142, 171.6227766016838245, 27.69059892324149530 ) ) ;
#13646=DIRECTION ( 'NONE',  ( 1.000000000000000000, -0.000000000000000000, -0.000000000000000000 ) ) ;
#13782=ORIENTED_EDGE ( 'NONE', *, *, #16757, .T. ) ;
#13833=DIRECTION ( 'NONE',  ( 1.000000000000000000, -0.000000000000000000, -0.000000000000000000 ) ) ;
#13851=DIRECTION ( 'NONE',  ( 0.000000000000000000, 0.000000000000000000, -1.000000000000000000 ) ) ;
#14014=EDGE_LOOP ( 'NONE', ( #4363, #1137, #13365, #8676 ) ) ;
#14017=FACE_BOUND ( 'NONE', #4129, .T. ) ;
#14052=ORIENTED_EDGE ( 'NONE', *, *, #10792, .T. ) ;
#14099=CARTESIAN_POINT ( 'NONE',  ( -116.4755503550297107, 171.6227766016838245, 0.000000000000000000 ) ) ;
#14165=AXIS2_PLACEMENT_3D ( 'NONE', #6967, #5644, #16455 ) ;
#14197=EDGE_CURVE ( 'NONE', #16730, #1036, #2501, .T. ) ;
#14226=ORIENTED_EDGE ( 'NONE', *, *, #13390, .F. ) ;
#14229=DIRECTION ( 'NONE',  ( 0.000000000000000000, 1.000000000000000000, -1.224646799147353207E-16 ) ) ;
#14240=CARTESIAN_POINT ( 'NONE',  ( -153.0000000000000284, 171.6227766016838245, 23.57392898041431195 ) ) ;
#14282=AXIS2_PLACEMENT_3D ( 'NONE', #724, #6117, #972 ) ;
#14468=ORIENTED_EDGE ( 'NONE', *, *, #12250, .T. ) ;
#14490=EDGE_LOOP ( 'NONE', ( #14226, #9855 ) ) ;
#14500=DIRECTION ( 'NONE',  ( 0.000000000000000000, 0.000000000000000000, -1.000000000000000000 ) ) ;
#14701=CARTESIAN_POINT ( 'NONE',  ( -151.0000000000000284, 171.6227766016838245, 0.000000000000000000 ) ) ;
#14829=AXIS2_PLACEMENT_3D ( 'NONE', #641, #8331, #7104 ) ;
#14895=AXIS2_PLACEMENT_3D ( 'NONE', #6177, #4769, #4854 ) ;
#14938=DIRECTION ( 'NONE',  ( 1.000000000000000000, -0.000000000000000000, -0.000000000000000000 ) ) ;
#15114=EDGE_CURVE ( 'NONE', #2291, #13060, #16093, .T. ) ;
#15123=COLOUR_RGB ( '', 0.66274510, 0.83137255, 0.94901961) ;
#15134=FACE_OUTER_BOUND ( 'NONE', #13382, .T. ) ;
#15147=CIRCLE ( 'NONE', #17420, 23.57392898041429774 ) ;
#15150=AXIS2_PLACEMENT_3D ( 'NONE', #9755, #16331, #5520 ) ;
#15183=ORIENTED_EDGE ( 'NONE', *, *, #9928, .F. ) ;
#15196=PRODUCT_DEFINITION_FORMATION_WITH_SPECIFIED_SOURCE ( 'ANY', '', #3197, .NOT_KNOWN. ) ;
#15286=( NAMED_UNIT ( * ) SI_UNIT ( $, .STERADIAN. ) SOLID_ANGLE_UNIT ( ) );
#15318=CARTESIAN_POINT ( 'NONE',  ( -100.0000000000000000, 171.6227766016838245, -27.69059892324149530 ) ) ;
#15328=FACE_OUTER_BOUND ( 'NONE', #2275, .T. ) ;
#15418=ORIENTED_EDGE ( 'NONE', *, *, #4925, .T. ) ;
#15473=EDGE_LOOP ( 'NONE', ( #1994, #7739 ) ) ;
#15504=DIRECTION ( 'NONE',  ( 0.000000000000000000, 0.000000000000000000, -1.000000000000000000 ) ) ;
#15538=ORIENTED_EDGE ( 'NONE', *, *, #10399, .F. ) ;
#15632=CARTESIAN_POINT ( 'NONE',  ( -151.6393416600920716, 171.6227766016838245, 25.46898629924947244 ) ) ;
#15669=CIRCLE ( 'NONE', #13419, 25.46898629924947244 ) ;
#15677=PLANE ( 'NONE',  #12325 ) ;
#15679=DIRECTION ( 'NONE',  ( 0.000000000000000000, 1.000000000000000000, 1.224646799147353207E-16 ) ) ;
#15736=MECHANICAL_DESIGN_GEOMETRIC_PRESENTATION_REPRESENTATION('',(#2461),#10934);
#15781=CARTESIAN_POINT ( 'NONE',  ( -151.0000000000000284, 171.6227766016838245, 0.000000000000000000 ) ) ;
#15795=AXIS2_PLACEMENT_3D ( 'NONE', #13349, #15995, #6337 ) ;
#15814=VERTEX_POINT ( 'NONE', #4914 ) ;
#15874=DIRECTION ( 'NONE',  ( 1.000000000000000000, -0.000000000000000000, -0.000000000000000000 ) ) ;
#15968=CIRCLE ( 'NONE', #14829, 23.57392898041431195 ) ;
#15995=DIRECTION ( 'NONE',  ( 1.000000000000000000, 0.000000000000000000, -0.000000000000000000 ) ) ;
#15997=FACE_OUTER_BOUND ( 'NONE', #16044, .T. ) ;
#16007=CIRCLE ( 'NONE', #15150, 25.69059892324149175 ) ;
#16013=ORIENTED_EDGE ( 'NONE', *, *, #3322, .T. ) ;
#16019=TOROIDAL_SURFACE ( 'NONE', #11209, -78.75916623668499028, 108.0000000000000142 ) ;
#16044=EDGE_LOOP ( 'NONE', ( #2942, #10521, #4834, #11686 ) ) ;
#16093=CIRCLE ( 'NONE', #9876, 27.69059892324149530 ) ;
#16108=DIRECTION ( 'NONE',  ( 1.000000000000000000, -0.000000000000000000, -0.000000000000000000 ) ) ;
#16114=CARTESIAN_POINT ( 'NONE',  ( -103.0000000000000142, 171.6227766016838245, 0.000000000000000000 ) ) ;
#16125=VECTOR ( 'NONE', #3357, 1000.000000000000000 ) ;
#16145=ORIENTED_EDGE ( 'NONE', *, *, #7134, .F. ) ;
#16146=CARTESIAN_POINT ( 'NONE',  ( -95.00000000000000000, 171.6227766016838245, -27.69059892324149530 ) ) ;
#16163=EDGE_CURVE ( 'NONE', #5246, #6881, #3233, .T. ) ;
#16198=EDGE_CURVE ( 'NONE', #8608, #5246, #11998, .T. ) ;
#16248=DIRECTION ( 'NONE',  ( -0.000000000000000000, -1.000000000000000000, -0.000000000000000000 ) ) ;
#16312=ORIENTED_EDGE ( 'NONE', *, *, #3605, .F. ) ;
#16314=EDGE_LOOP ( 'NONE', ( #996, #959, #1821, #45 ) ) ;
#16321=CARTESIAN_POINT ( 'NONE',  ( -102.0000000000000142, 171.6227766016838245, 28.26633746182137585 ) ) ;
#16331=DIRECTION ( 'NONE',  ( 1.000000000000000000, -0.000000000000000000, -0.000000000000000000 ) ) ;
#16341=DIRECTION ( 'NONE',  ( -1.000000000000000000, 0.000000000000000000, 0.000000000000000000 ) ) ;
#16359=EDGE_CURVE ( 'NONE', #16418, #5242, #11142, .T. ) ;
#16368=EDGE_CURVE ( 'NONE', #8608, #10629, #15669, .T. ) ;
#16412=AXIS2_PLACEMENT_3D ( 'NONE', #691, #9974, #6085 ) ;
#16418=VERTEX_POINT ( 'NONE', #10260 ) ;
#16428=EDGE_CURVE ( 'NONE', #3610, #5121, #6411, .T. ) ;
#16455=DIRECTION ( 'NONE',  ( 0.000000000000000000, 0.000000000000000000, -1.000000000000000000 ) ) ;
#16575=DIRECTION ( 'NONE',  ( 0.000000000000000000, 0.000000000000000000, -1.000000000000000000 ) ) ;
#16676=DIRECTION ( 'NONE',  ( 1.000000000000000000, -0.000000000000000000, -0.000000000000000000 ) ) ;
#16690=AXIS2_PLACEMENT_3D ( 'NONE', #6342, #17415, #9089 ) ;
#16708=EDGE_CURVE ( 'NONE', #10629, #6881, #1028, .T. ) ;
#16725=( NAMED_UNIT ( * ) PLANE_ANGLE_UNIT ( ) SI_UNIT ( $, .RADIAN. ) );
#16730=VERTEX_POINT ( 'NONE', #16984 ) ;
#16738=DIRECTION ( 'NONE',  ( 1.000000000000000000, -0.000000000000000000, -0.000000000000000000 ) ) ;
#16757=EDGE_CURVE ( 'NONE', #13060, #2291, #2446, .T. ) ;
#16764=ORIENTED_EDGE ( 'NONE', *, *, #17060, .T. ) ;
#16785=DIRECTION ( 'NONE',  ( 0.000000000000000000, 0.000000000000000000, 1.000000000000000000 ) ) ;
#16877=PRESENTATION_STYLE_ASSIGNMENT (( #7477 ) ) ;
#16919=UNCERTAINTY_MEASURE_WITH_UNIT (LENGTH_MEASURE( 1.000000000000000082E-05 ), #12805, 'distance_accuracy_value', 'NONE');
#16984=CARTESIAN_POINT ( 'NONE',  ( -151.0000000000000284, 171.6227766016838245, 6.000000000000005329 ) ) ;
#16995=CARTESIAN_POINT ( 'NONE',  ( -151.0000000000000284, 171.6227766016838245, 0.000000000000000000 ) ) ;
#17016=ORIENTED_EDGE ( 'NONE', *, *, #146, .T. ) ;
#17020=DIRECTION ( 'NONE',  ( 0.000000000000000000, 1.000000000000000000, -1.224646799147353207E-16 ) ) ;
#17022=DIRECTION ( 'NONE',  ( -1.000000000000000000, 0.000000000000000000, 0.000000000000000000 ) ) ;
#17026=DIRECTION ( 'NONE',  ( 0.000000000000000000, 0.000000000000000000, -1.000000000000000000 ) ) ;
#17060=EDGE_CURVE ( 'NONE', #554, #2291, #1559, .T. ) ;
#17101=AXIS2_PLACEMENT_3D ( 'NONE', #3021, #4540, #15504 ) ;
#17121=ORIENTED_EDGE ( 'NONE', *, *, #16359, .F. ) ;
#17147=CARTESIAN_POINT ( 'NONE',  ( -153.0000000000000284, 171.6227766016838245, -23.57392898041431195 ) ) ;
#17180=CYLINDRICAL_SURFACE ( 'NONE', #9173, 27.69059892324149530 ) ;
#17369=VECTOR ( 'NONE', #7552, 1000.000000000000000 ) ;
#17383=VERTEX_POINT ( 'NONE', #11853 ) ;
#17415=DIRECTION ( 'NONE',  ( -1.000000000000000000, 0.000000000000000000, 0.000000000000000000 ) ) ;
#17420=AXIS2_PLACEMENT_3D ( 'NONE', #15781, #15874, #17026 ) ;
#17428=CARTESIAN_POINT ( 'NONE',  ( -151.0000000000000284, 171.6227766016838245, 0.000000000000000000 ) ) ;
#17460=ORIENTED_EDGE ( 'NONE', *, *, #13390, .T. ) ;
ENDSEC;
END-ISO-10303-21;
